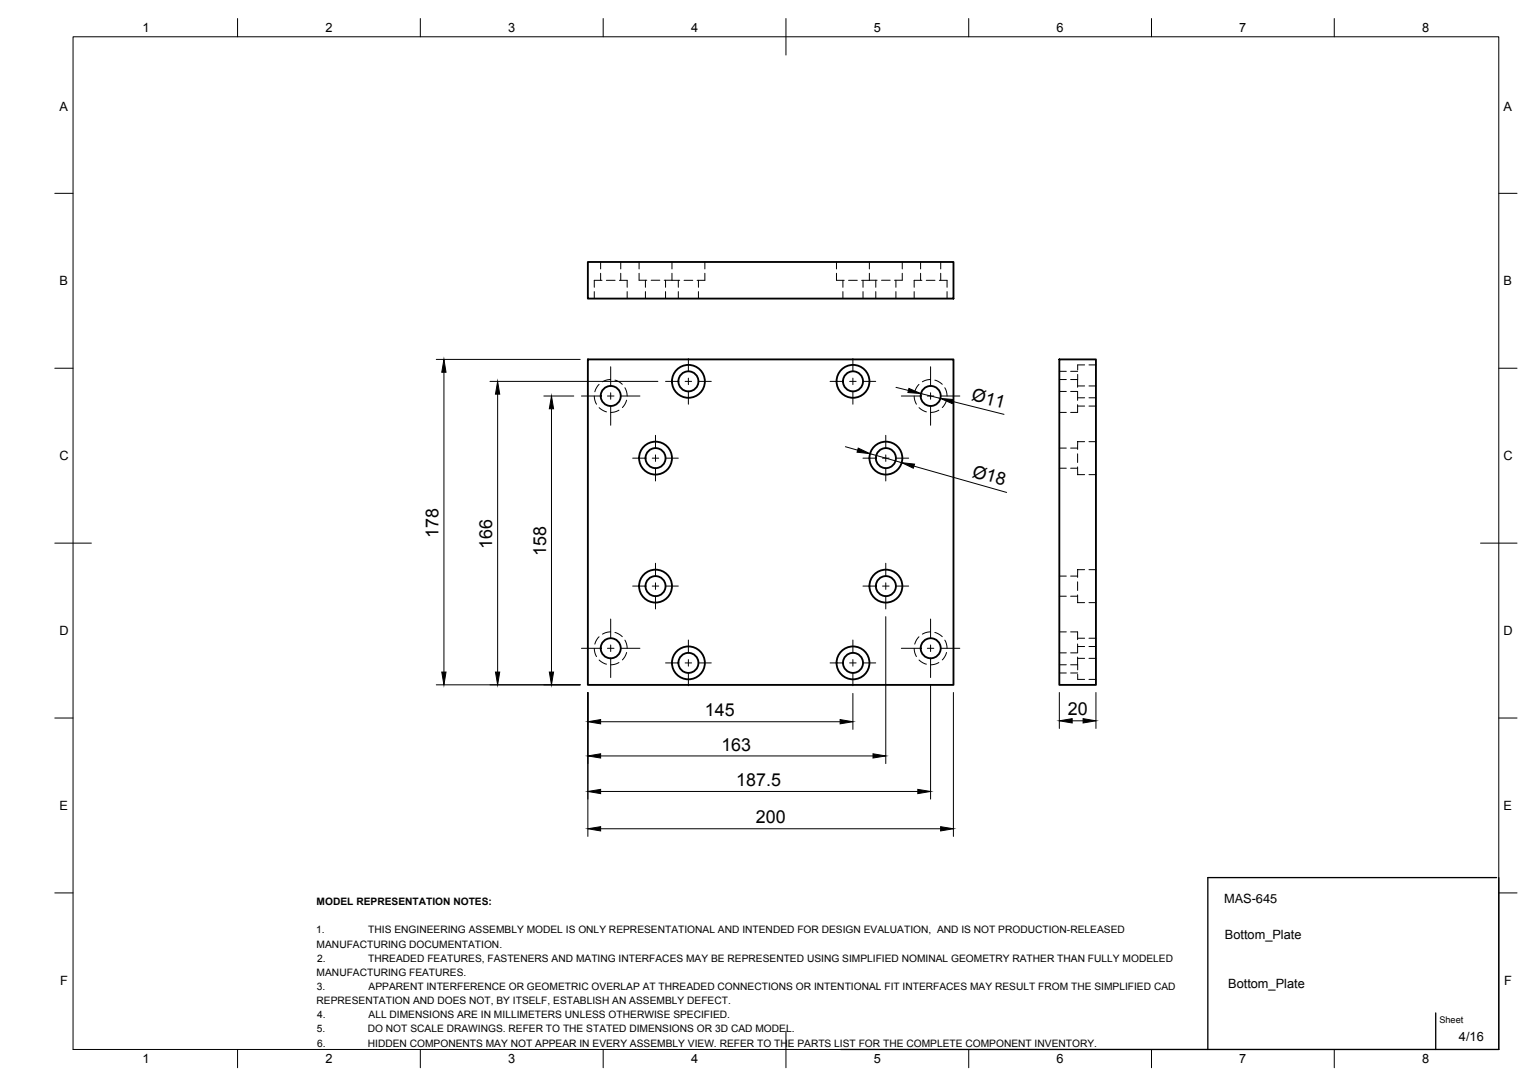
ISO-10303-21;
HEADER;
FILE_DESCRIPTION((''),'2;1');
FILE_NAME('Bottom_Plate.step','2026-10-09T10:54:55-07:00',(''),(''),'','','');
FILE_SCHEMA (('AUTOMOTIVE_DESIGN { 1 0 10303 214 3 1 1 }'));
ENDSEC;
DATA;
#10=MECHANICAL_DESIGN_GEOMETRIC_PRESENTATION_REPRESENTATION('',(#596),#63824);
#566=SHAPE_REPRESENTATION_RELATIONSHIP('SRR','None',#63880,#581) ;
#581=ADVANCED_BREP_SHAPE_REPRESENTATION('',(#611),#63810) ;
#596=STYLED_ITEM('',(#63963),#611) ;
#611=MANIFOLD_SOLID_BREP('Body1',#15495) ;
#651=FACE_BOUND('',#2476,.T.) ;
#652=FACE_BOUND('',#2480,.T.) ;
#653=FACE_BOUND('',#2484,.T.) ;
#654=FACE_BOUND('',#2488,.T.) ;
#655=FACE_BOUND('',#2492,.T.) ;
#656=FACE_BOUND('',#2496,.T.) ;
#657=FACE_BOUND('',#2500,.T.) ;
#658=FACE_BOUND('',#2504,.T.) ;
#659=FACE_BOUND('',#2508,.T.) ;
#660=FACE_BOUND('',#2512,.T.) ;
#661=FACE_BOUND('',#2516,.T.) ;
#662=FACE_BOUND('',#2520,.T.) ;
#663=FACE_BOUND('',#2524,.T.) ;
#664=FACE_BOUND('',#2525,.T.) ;
#665=FACE_BOUND('',#2526,.T.) ;
#666=FACE_BOUND('',#2527,.T.) ;
#667=FACE_BOUND('',#2528,.T.) ;
#668=FACE_BOUND('',#2529,.T.) ;
#669=FACE_BOUND('',#2530,.T.) ;
#670=FACE_BOUND('',#2531,.T.) ;
#671=FACE_BOUND('',#2532,.T.) ;
#672=FACE_BOUND('',#2533,.T.) ;
#673=FACE_BOUND('',#2534,.T.) ;
#674=FACE_BOUND('',#2535,.T.) ;
#675=FACE_BOUND('',#2538,.T.) ;
#676=FACE_BOUND('',#2539,.T.) ;
#677=FACE_BOUND('',#2540,.T.) ;
#678=FACE_BOUND('',#2541,.T.) ;
#679=FACE_BOUND('',#2542,.T.) ;
#680=FACE_BOUND('',#2543,.T.) ;
#681=FACE_BOUND('',#2544,.T.) ;
#682=FACE_BOUND('',#2545,.T.) ;
#683=FACE_BOUND('',#2546,.T.) ;
#684=FACE_BOUND('',#2547,.T.) ;
#685=FACE_BOUND('',#2548,.T.) ;
#686=FACE_BOUND('',#2549,.T.) ;
#842=PLANE('',#15763) ;
#843=PLANE('',#15770) ;
#844=PLANE('',#15777) ;
#845=PLANE('',#15784) ;
#846=PLANE('',#15791) ;
#847=PLANE('',#15798) ;
#848=PLANE('',#15805) ;
#849=PLANE('',#15812) ;
#850=PLANE('',#15819) ;
#851=PLANE('',#15826) ;
#852=PLANE('',#15833) ;
#853=PLANE('',#15840) ;
#854=PLANE('',#15847) ;
#855=PLANE('',#15848) ;
#856=PLANE('',#15849) ;
#857=PLANE('',#15850) ;
#858=PLANE('',#15851) ;
#859=PLANE('',#15852) ;
#1137=CYLINDRICAL_SURFACE('',#15766,9.) ;
#1138=CYLINDRICAL_SURFACE('',#15768,5.5) ;
#1139=CYLINDRICAL_SURFACE('',#15773,9.) ;
#1140=CYLINDRICAL_SURFACE('',#15775,5.5) ;
#1141=CYLINDRICAL_SURFACE('',#15780,9.) ;
#1142=CYLINDRICAL_SURFACE('',#15782,5.5) ;
#1143=CYLINDRICAL_SURFACE('',#15787,9.) ;
#1144=CYLINDRICAL_SURFACE('',#15789,5.5) ;
#1145=CYLINDRICAL_SURFACE('',#15794,9.) ;
#1146=CYLINDRICAL_SURFACE('',#15796,5.5) ;
#1147=CYLINDRICAL_SURFACE('',#15801,9.) ;
#1148=CYLINDRICAL_SURFACE('',#15803,5.5) ;
#1149=CYLINDRICAL_SURFACE('',#15808,9.) ;
#1150=CYLINDRICAL_SURFACE('',#15810,5.5) ;
#1151=CYLINDRICAL_SURFACE('',#15815,9.) ;
#1152=CYLINDRICAL_SURFACE('',#15817,5.5) ;
#1153=CYLINDRICAL_SURFACE('',#15822,9.) ;
#1154=CYLINDRICAL_SURFACE('',#15824,5.5) ;
#1155=CYLINDRICAL_SURFACE('',#15829,9.) ;
#1156=CYLINDRICAL_SURFACE('',#15831,5.5) ;
#1157=CYLINDRICAL_SURFACE('',#15836,9.) ;
#1158=CYLINDRICAL_SURFACE('',#15838,5.5) ;
#1159=CYLINDRICAL_SURFACE('',#15843,9.) ;
#1160=CYLINDRICAL_SURFACE('',#15845,5.5) ;
#1588=FACE_OUTER_BOUND('',#2475,.T.) ;
#1589=FACE_OUTER_BOUND('',#2477,.T.) ;
#1590=FACE_OUTER_BOUND('',#2478,.T.) ;
#1591=FACE_OUTER_BOUND('',#2479,.T.) ;
#1592=FACE_OUTER_BOUND('',#2481,.T.) ;
#1593=FACE_OUTER_BOUND('',#2482,.T.) ;
#1594=FACE_OUTER_BOUND('',#2483,.T.) ;
#1595=FACE_OUTER_BOUND('',#2485,.T.) ;
#1596=FACE_OUTER_BOUND('',#2486,.T.) ;
#1597=FACE_OUTER_BOUND('',#2487,.T.) ;
#1598=FACE_OUTER_BOUND('',#2489,.T.) ;
#1599=FACE_OUTER_BOUND('',#2490,.T.) ;
#1600=FACE_OUTER_BOUND('',#2491,.T.) ;
#1601=FACE_OUTER_BOUND('',#2493,.T.) ;
#1602=FACE_OUTER_BOUND('',#2494,.T.) ;
#1603=FACE_OUTER_BOUND('',#2495,.T.) ;
#1604=FACE_OUTER_BOUND('',#2497,.T.) ;
#1605=FACE_OUTER_BOUND('',#2498,.T.) ;
#1606=FACE_OUTER_BOUND('',#2499,.T.) ;
#1607=FACE_OUTER_BOUND('',#2501,.T.) ;
#1608=FACE_OUTER_BOUND('',#2502,.T.) ;
#1609=FACE_OUTER_BOUND('',#2503,.T.) ;
#1610=FACE_OUTER_BOUND('',#2505,.T.) ;
#1611=FACE_OUTER_BOUND('',#2506,.T.) ;
#1612=FACE_OUTER_BOUND('',#2507,.T.) ;
#1613=FACE_OUTER_BOUND('',#2509,.T.) ;
#1614=FACE_OUTER_BOUND('',#2510,.T.) ;
#1615=FACE_OUTER_BOUND('',#2511,.T.) ;
#1616=FACE_OUTER_BOUND('',#2513,.T.) ;
#1617=FACE_OUTER_BOUND('',#2514,.T.) ;
#1618=FACE_OUTER_BOUND('',#2515,.T.) ;
#1619=FACE_OUTER_BOUND('',#2517,.T.) ;
#1620=FACE_OUTER_BOUND('',#2518,.T.) ;
#1621=FACE_OUTER_BOUND('',#2519,.T.) ;
#1622=FACE_OUTER_BOUND('',#2521,.T.) ;
#1623=FACE_OUTER_BOUND('',#2522,.T.) ;
#1624=FACE_OUTER_BOUND('',#2523,.T.) ;
#1625=FACE_OUTER_BOUND('',#2536,.T.) ;
#1626=FACE_OUTER_BOUND('',#2537,.T.) ;
#1627=FACE_OUTER_BOUND('',#2550,.T.) ;
#1628=FACE_OUTER_BOUND('',#2551,.T.) ;
#1629=FACE_OUTER_BOUND('',#2552,.T.) ;
#2475=EDGE_LOOP('',(#9976)) ;
#2476=EDGE_LOOP('',(#9977)) ;
#2477=EDGE_LOOP('',(#9978,#9979,#9980,#9981)) ;
#2478=EDGE_LOOP('',(#9982,#9983,#9984,#9985)) ;
#2479=EDGE_LOOP('',(#9986)) ;
#2480=EDGE_LOOP('',(#9987)) ;
#2481=EDGE_LOOP('',(#9988,#9989,#9990,#9991)) ;
#2482=EDGE_LOOP('',(#9992,#9993,#9994,#9995)) ;
#2483=EDGE_LOOP('',(#9996)) ;
#2484=EDGE_LOOP('',(#9997)) ;
#2485=EDGE_LOOP('',(#9998,#9999,#10000,#10001)) ;
#2486=EDGE_LOOP('',(#10002,#10003,#10004,#10005)) ;
#2487=EDGE_LOOP('',(#10006)) ;
#2488=EDGE_LOOP('',(#10007)) ;
#2489=EDGE_LOOP('',(#10008,#10009,#10010,#10011)) ;
#2490=EDGE_LOOP('',(#10012,#10013,#10014,#10015)) ;
#2491=EDGE_LOOP('',(#10016)) ;
#2492=EDGE_LOOP('',(#10017)) ;
#2493=EDGE_LOOP('',(#10018,#10019,#10020,#10021)) ;
#2494=EDGE_LOOP('',(#10022,#10023,#10024,#10025)) ;
#2495=EDGE_LOOP('',(#10026)) ;
#2496=EDGE_LOOP('',(#10027)) ;
#2497=EDGE_LOOP('',(#10028,#10029,#10030,#10031)) ;
#2498=EDGE_LOOP('',(#10032,#10033,#10034,#10035)) ;
#2499=EDGE_LOOP('',(#10036)) ;
#2500=EDGE_LOOP('',(#10037)) ;
#2501=EDGE_LOOP('',(#10038,#10039,#10040,#10041)) ;
#2502=EDGE_LOOP('',(#10042,#10043,#10044,#10045)) ;
#2503=EDGE_LOOP('',(#10046)) ;
#2504=EDGE_LOOP('',(#10047)) ;
#2505=EDGE_LOOP('',(#10048,#10049,#10050,#10051)) ;
#2506=EDGE_LOOP('',(#10052,#10053,#10054,#10055)) ;
#2507=EDGE_LOOP('',(#10056)) ;
#2508=EDGE_LOOP('',(#10057)) ;
#2509=EDGE_LOOP('',(#10058,#10059,#10060,#10061)) ;
#2510=EDGE_LOOP('',(#10062,#10063,#10064,#10065)) ;
#2511=EDGE_LOOP('',(#10066)) ;
#2512=EDGE_LOOP('',(#10067)) ;
#2513=EDGE_LOOP('',(#10068,#10069,#10070,#10071)) ;
#2514=EDGE_LOOP('',(#10072,#10073,#10074,#10075)) ;
#2515=EDGE_LOOP('',(#10076)) ;
#2516=EDGE_LOOP('',(#10077)) ;
#2517=EDGE_LOOP('',(#10078,#10079,#10080,#10081)) ;
#2518=EDGE_LOOP('',(#10082,#10083,#10084,#10085)) ;
#2519=EDGE_LOOP('',(#10086)) ;
#2520=EDGE_LOOP('',(#10087)) ;
#2521=EDGE_LOOP('',(#10088,#10089,#10090,#10091)) ;
#2522=EDGE_LOOP('',(#10092,#10093,#10094,#10095)) ;
#2523=EDGE_LOOP('',(#10096,#10097,#10098,#10099)) ;
#2524=EDGE_LOOP('',(#10100)) ;
#2525=EDGE_LOOP('',(#10101)) ;
#2526=EDGE_LOOP('',(#10102)) ;
#2527=EDGE_LOOP('',(#10103)) ;
#2528=EDGE_LOOP('',(#10104)) ;
#2529=EDGE_LOOP('',(#10105)) ;
#2530=EDGE_LOOP('',(#10106)) ;
#2531=EDGE_LOOP('',(#10107)) ;
#2532=EDGE_LOOP('',(#10108)) ;
#2533=EDGE_LOOP('',(#10109)) ;
#2534=EDGE_LOOP('',(#10110)) ;
#2535=EDGE_LOOP('',(#10111)) ;
#2536=EDGE_LOOP('',(#10112,#10113,#10114,#10115)) ;
#2537=EDGE_LOOP('',(#10116,#10117,#10118,#10119)) ;
#2538=EDGE_LOOP('',(#10120)) ;
#2539=EDGE_LOOP('',(#10121)) ;
#2540=EDGE_LOOP('',(#10122)) ;
#2541=EDGE_LOOP('',(#10123)) ;
#2542=EDGE_LOOP('',(#10124)) ;
#2543=EDGE_LOOP('',(#10125)) ;
#2544=EDGE_LOOP('',(#10126)) ;
#2545=EDGE_LOOP('',(#10127)) ;
#2546=EDGE_LOOP('',(#10128)) ;
#2547=EDGE_LOOP('',(#10129)) ;
#2548=EDGE_LOOP('',(#10130)) ;
#2549=EDGE_LOOP('',(#10131)) ;
#2550=EDGE_LOOP('',(#10132,#10133,#10134,#10135)) ;
#2551=EDGE_LOOP('',(#10136,#10137,#10138,#10139)) ;
#2552=EDGE_LOOP('',(#10140,#10141,#10142,#10143)) ;
#3516=CIRCLE('',#15764,9.) ;
#3517=CIRCLE('',#15765,5.5) ;
#3518=CIRCLE('',#15767,9.) ;
#3519=CIRCLE('',#15769,5.5) ;
#3520=CIRCLE('',#15771,9.) ;
#3521=CIRCLE('',#15772,5.5) ;
#3522=CIRCLE('',#15774,9.) ;
#3523=CIRCLE('',#15776,5.5) ;
#3524=CIRCLE('',#15778,9.) ;
#3525=CIRCLE('',#15779,5.5) ;
#3526=CIRCLE('',#15781,9.) ;
#3527=CIRCLE('',#15783,5.5) ;
#3528=CIRCLE('',#15785,9.) ;
#3529=CIRCLE('',#15786,5.5) ;
#3530=CIRCLE('',#15788,9.) ;
#3531=CIRCLE('',#15790,5.5) ;
#3532=CIRCLE('',#15792,9.) ;
#3533=CIRCLE('',#15793,5.5) ;
#3534=CIRCLE('',#15795,9.) ;
#3535=CIRCLE('',#15797,5.5) ;
#3536=CIRCLE('',#15799,9.) ;
#3537=CIRCLE('',#15800,5.5) ;
#3538=CIRCLE('',#15802,9.) ;
#3539=CIRCLE('',#15804,5.5) ;
#3540=CIRCLE('',#15806,9.) ;
#3541=CIRCLE('',#15807,5.5) ;
#3542=CIRCLE('',#15809,9.) ;
#3543=CIRCLE('',#15811,5.5) ;
#3544=CIRCLE('',#15813,9.) ;
#3545=CIRCLE('',#15814,5.5) ;
#3546=CIRCLE('',#15816,9.) ;
#3547=CIRCLE('',#15818,5.5) ;
#3548=CIRCLE('',#15820,9.) ;
#3549=CIRCLE('',#15821,5.5) ;
#3550=CIRCLE('',#15823,9.) ;
#3551=CIRCLE('',#15825,5.5) ;
#3552=CIRCLE('',#15827,9.) ;
#3553=CIRCLE('',#15828,5.5) ;
#3554=CIRCLE('',#15830,9.) ;
#3555=CIRCLE('',#15832,5.5) ;
#3556=CIRCLE('',#15834,9.) ;
#3557=CIRCLE('',#15835,5.5) ;
#3558=CIRCLE('',#15837,9.) ;
#3559=CIRCLE('',#15839,5.5) ;
#3560=CIRCLE('',#15841,9.) ;
#3561=CIRCLE('',#15842,5.5) ;
#3562=CIRCLE('',#15844,9.) ;
#3563=CIRCLE('',#15846,5.5) ;
#4735=LINE('',#23215,#5391) ;
#4736=LINE('',#23218,#5392) ;
#4737=LINE('',#23228,#5393) ;
#4738=LINE('',#23231,#5394) ;
#4739=LINE('',#23241,#5395) ;
#4740=LINE('',#23244,#5396) ;
#4741=LINE('',#23254,#5397) ;
#4742=LINE('',#23257,#5398) ;
#4743=LINE('',#23267,#5399) ;
#4744=LINE('',#23270,#5400) ;
#4745=LINE('',#23280,#5401) ;
#4746=LINE('',#23283,#5402) ;
#4747=LINE('',#23293,#5403) ;
#4748=LINE('',#23296,#5404) ;
#4749=LINE('',#23306,#5405) ;
#4750=LINE('',#23309,#5406) ;
#4751=LINE('',#23319,#5407) ;
#4752=LINE('',#23322,#5408) ;
#4753=LINE('',#23332,#5409) ;
#4754=LINE('',#23335,#5410) ;
#4755=LINE('',#23345,#5411) ;
#4756=LINE('',#23348,#5412) ;
#4757=LINE('',#23358,#5413) ;
#4758=LINE('',#23361,#5414) ;
#4759=LINE('',#23366,#5415) ;
#4760=LINE('',#23368,#5416) ;
#4761=LINE('',#23370,#5417) ;
#4762=LINE('',#23371,#5418) ;
#4763=LINE('',#23374,#5419) ;
#4764=LINE('',#23376,#5420) ;
#4765=LINE('',#23377,#5421) ;
#4766=LINE('',#23380,#5422) ;
#4767=LINE('',#23382,#5423) ;
#4768=LINE('',#23383,#5424) ;
#4769=LINE('',#23385,#5425) ;
#4770=LINE('',#23386,#5426) ;
#5391=VECTOR('',#18133,9.) ;
#5392=VECTOR('',#18136,5.5) ;
#5393=VECTOR('',#18149,9.) ;
#5394=VECTOR('',#18152,5.5) ;
#5395=VECTOR('',#18165,9.) ;
#5396=VECTOR('',#18168,5.5) ;
#5397=VECTOR('',#18181,9.) ;
#5398=VECTOR('',#18184,5.5) ;
#5399=VECTOR('',#18197,9.) ;
#5400=VECTOR('',#18200,5.5) ;
#5401=VECTOR('',#18213,9.) ;
#5402=VECTOR('',#18216,5.5) ;
#5403=VECTOR('',#18229,9.) ;
#5404=VECTOR('',#18232,5.5) ;
#5405=VECTOR('',#18245,9.) ;
#5406=VECTOR('',#18248,5.5) ;
#5407=VECTOR('',#18261,9.) ;
#5408=VECTOR('',#18264,5.5) ;
#5409=VECTOR('',#18277,9.) ;
#5410=VECTOR('',#18280,5.5) ;
#5411=VECTOR('',#18293,9.) ;
#5412=VECTOR('',#18296,5.5) ;
#5413=VECTOR('',#18309,9.) ;
#5414=VECTOR('',#18312,5.5) ;
#5415=VECTOR('',#18317,10.) ;
#5416=VECTOR('',#18318,10.) ;
#5417=VECTOR('',#18319,10.) ;
#5418=VECTOR('',#18320,10.) ;
#5419=VECTOR('',#18323,10.) ;
#5420=VECTOR('',#18324,10.) ;
#5421=VECTOR('',#18325,10.) ;
#5422=VECTOR('',#18328,10.) ;
#5423=VECTOR('',#18329,10.) ;
#5424=VECTOR('',#18330,10.) ;
#5425=VECTOR('',#18333,10.) ;
#5426=VECTOR('',#18334,10.) ;
#6064=VERTEX_POINT('',#23208) ;
#6065=VERTEX_POINT('',#23210) ;
#6066=VERTEX_POINT('',#23213) ;
#6067=VERTEX_POINT('',#23217) ;
#6068=VERTEX_POINT('',#23221) ;
#6069=VERTEX_POINT('',#23223) ;
#6070=VERTEX_POINT('',#23226) ;
#6071=VERTEX_POINT('',#23230) ;
#6072=VERTEX_POINT('',#23234) ;
#6073=VERTEX_POINT('',#23236) ;
#6074=VERTEX_POINT('',#23239) ;
#6075=VERTEX_POINT('',#23243) ;
#6076=VERTEX_POINT('',#23247) ;
#6077=VERTEX_POINT('',#23249) ;
#6078=VERTEX_POINT('',#23252) ;
#6079=VERTEX_POINT('',#23256) ;
#6080=VERTEX_POINT('',#23260) ;
#6081=VERTEX_POINT('',#23262) ;
#6082=VERTEX_POINT('',#23265) ;
#6083=VERTEX_POINT('',#23269) ;
#6084=VERTEX_POINT('',#23273) ;
#6085=VERTEX_POINT('',#23275) ;
#6086=VERTEX_POINT('',#23278) ;
#6087=VERTEX_POINT('',#23282) ;
#6088=VERTEX_POINT('',#23286) ;
#6089=VERTEX_POINT('',#23288) ;
#6090=VERTEX_POINT('',#23291) ;
#6091=VERTEX_POINT('',#23295) ;
#6092=VERTEX_POINT('',#23299) ;
#6093=VERTEX_POINT('',#23301) ;
#6094=VERTEX_POINT('',#23304) ;
#6095=VERTEX_POINT('',#23308) ;
#6096=VERTEX_POINT('',#23312) ;
#6097=VERTEX_POINT('',#23314) ;
#6098=VERTEX_POINT('',#23317) ;
#6099=VERTEX_POINT('',#23321) ;
#6100=VERTEX_POINT('',#23325) ;
#6101=VERTEX_POINT('',#23327) ;
#6102=VERTEX_POINT('',#23330) ;
#6103=VERTEX_POINT('',#23334) ;
#6104=VERTEX_POINT('',#23338) ;
#6105=VERTEX_POINT('',#23340) ;
#6106=VERTEX_POINT('',#23343) ;
#6107=VERTEX_POINT('',#23347) ;
#6108=VERTEX_POINT('',#23351) ;
#6109=VERTEX_POINT('',#23353) ;
#6110=VERTEX_POINT('',#23356) ;
#6111=VERTEX_POINT('',#23360) ;
#6112=VERTEX_POINT('',#23364) ;
#6113=VERTEX_POINT('',#23365) ;
#6114=VERTEX_POINT('',#23367) ;
#6115=VERTEX_POINT('',#23369) ;
#6116=VERTEX_POINT('',#23373) ;
#6117=VERTEX_POINT('',#23375) ;
#6118=VERTEX_POINT('',#23379) ;
#6119=VERTEX_POINT('',#23381) ;
#7542=EDGE_CURVE('',#6064,#6064,#3516,.T.) ;
#7543=EDGE_CURVE('',#6065,#6065,#3517,.T.) ;
#7544=EDGE_CURVE('',#6066,#6066,#3518,.T.) ;
#7545=EDGE_CURVE('',#6066,#6064,#4735,.T.) ;
#7546=EDGE_CURVE('',#6065,#6067,#4736,.T.) ;
#7547=EDGE_CURVE('',#6067,#6067,#3519,.T.) ;
#7548=EDGE_CURVE('',#6068,#6068,#3520,.T.) ;
#7549=EDGE_CURVE('',#6069,#6069,#3521,.T.) ;
#7550=EDGE_CURVE('',#6070,#6070,#3522,.T.) ;
#7551=EDGE_CURVE('',#6070,#6068,#4737,.T.) ;
#7552=EDGE_CURVE('',#6069,#6071,#4738,.T.) ;
#7553=EDGE_CURVE('',#6071,#6071,#3523,.T.) ;
#7554=EDGE_CURVE('',#6072,#6072,#3524,.T.) ;
#7555=EDGE_CURVE('',#6073,#6073,#3525,.T.) ;
#7556=EDGE_CURVE('',#6074,#6074,#3526,.T.) ;
#7557=EDGE_CURVE('',#6074,#6072,#4739,.T.) ;
#7558=EDGE_CURVE('',#6073,#6075,#4740,.T.) ;
#7559=EDGE_CURVE('',#6075,#6075,#3527,.T.) ;
#7560=EDGE_CURVE('',#6076,#6076,#3528,.T.) ;
#7561=EDGE_CURVE('',#6077,#6077,#3529,.T.) ;
#7562=EDGE_CURVE('',#6078,#6078,#3530,.T.) ;
#7563=EDGE_CURVE('',#6078,#6076,#4741,.T.) ;
#7564=EDGE_CURVE('',#6077,#6079,#4742,.T.) ;
#7565=EDGE_CURVE('',#6079,#6079,#3531,.T.) ;
#7566=EDGE_CURVE('',#6080,#6080,#3532,.T.) ;
#7567=EDGE_CURVE('',#6081,#6081,#3533,.T.) ;
#7568=EDGE_CURVE('',#6082,#6082,#3534,.T.) ;
#7569=EDGE_CURVE('',#6082,#6080,#4743,.T.) ;
#7570=EDGE_CURVE('',#6081,#6083,#4744,.T.) ;
#7571=EDGE_CURVE('',#6083,#6083,#3535,.T.) ;
#7572=EDGE_CURVE('',#6084,#6084,#3536,.T.) ;
#7573=EDGE_CURVE('',#6085,#6085,#3537,.T.) ;
#7574=EDGE_CURVE('',#6086,#6086,#3538,.T.) ;
#7575=EDGE_CURVE('',#6086,#6084,#4745,.T.) ;
#7576=EDGE_CURVE('',#6085,#6087,#4746,.T.) ;
#7577=EDGE_CURVE('',#6087,#6087,#3539,.T.) ;
#7578=EDGE_CURVE('',#6088,#6088,#3540,.T.) ;
#7579=EDGE_CURVE('',#6089,#6089,#3541,.T.) ;
#7580=EDGE_CURVE('',#6090,#6090,#3542,.T.) ;
#7581=EDGE_CURVE('',#6090,#6088,#4747,.T.) ;
#7582=EDGE_CURVE('',#6089,#6091,#4748,.T.) ;
#7583=EDGE_CURVE('',#6091,#6091,#3543,.T.) ;
#7584=EDGE_CURVE('',#6092,#6092,#3544,.T.) ;
#7585=EDGE_CURVE('',#6093,#6093,#3545,.T.) ;
#7586=EDGE_CURVE('',#6094,#6094,#3546,.T.) ;
#7587=EDGE_CURVE('',#6094,#6092,#4749,.T.) ;
#7588=EDGE_CURVE('',#6093,#6095,#4750,.T.) ;
#7589=EDGE_CURVE('',#6095,#6095,#3547,.T.) ;
#7590=EDGE_CURVE('',#6096,#6096,#3548,.T.) ;
#7591=EDGE_CURVE('',#6097,#6097,#3549,.T.) ;
#7592=EDGE_CURVE('',#6098,#6098,#3550,.T.) ;
#7593=EDGE_CURVE('',#6098,#6096,#4751,.T.) ;
#7594=EDGE_CURVE('',#6097,#6099,#4752,.T.) ;
#7595=EDGE_CURVE('',#6099,#6099,#3551,.T.) ;
#7596=EDGE_CURVE('',#6100,#6100,#3552,.T.) ;
#7597=EDGE_CURVE('',#6101,#6101,#3553,.T.) ;
#7598=EDGE_CURVE('',#6102,#6102,#3554,.T.) ;
#7599=EDGE_CURVE('',#6102,#6100,#4753,.T.) ;
#7600=EDGE_CURVE('',#6101,#6103,#4754,.T.) ;
#7601=EDGE_CURVE('',#6103,#6103,#3555,.T.) ;
#7602=EDGE_CURVE('',#6104,#6104,#3556,.T.) ;
#7603=EDGE_CURVE('',#6105,#6105,#3557,.T.) ;
#7604=EDGE_CURVE('',#6106,#6106,#3558,.T.) ;
#7605=EDGE_CURVE('',#6106,#6104,#4755,.T.) ;
#7606=EDGE_CURVE('',#6105,#6107,#4756,.T.) ;
#7607=EDGE_CURVE('',#6107,#6107,#3559,.T.) ;
#7608=EDGE_CURVE('',#6108,#6108,#3560,.T.) ;
#7609=EDGE_CURVE('',#6109,#6109,#3561,.T.) ;
#7610=EDGE_CURVE('',#6110,#6110,#3562,.T.) ;
#7611=EDGE_CURVE('',#6110,#6108,#4757,.T.) ;
#7612=EDGE_CURVE('',#6109,#6111,#4758,.T.) ;
#7613=EDGE_CURVE('',#6111,#6111,#3563,.T.) ;
#7614=EDGE_CURVE('',#6112,#6113,#4759,.T.) ;
#7615=EDGE_CURVE('',#6114,#6113,#4760,.T.) ;
#7616=EDGE_CURVE('',#6114,#6115,#4761,.T.) ;
#7617=EDGE_CURVE('',#6115,#6112,#4762,.T.) ;
#7618=EDGE_CURVE('',#6113,#6116,#4763,.T.) ;
#7619=EDGE_CURVE('',#6117,#6116,#4764,.T.) ;
#7620=EDGE_CURVE('',#6117,#6114,#4765,.T.) ;
#7621=EDGE_CURVE('',#6116,#6118,#4766,.T.) ;
#7622=EDGE_CURVE('',#6119,#6118,#4767,.T.) ;
#7623=EDGE_CURVE('',#6119,#6117,#4768,.T.) ;
#7624=EDGE_CURVE('',#6118,#6112,#4769,.T.) ;
#7625=EDGE_CURVE('',#6115,#6119,#4770,.T.) ;
#9976=ORIENTED_EDGE('',*,*,#7542,.F.) ;
#9977=ORIENTED_EDGE('',*,*,#7543,.T.) ;
#9978=ORIENTED_EDGE('',*,*,#7544,.F.) ;
#9979=ORIENTED_EDGE('',*,*,#7545,.T.) ;
#9980=ORIENTED_EDGE('',*,*,#7542,.T.) ;
#9981=ORIENTED_EDGE('',*,*,#7545,.F.) ;
#9982=ORIENTED_EDGE('',*,*,#7543,.F.) ;
#9983=ORIENTED_EDGE('',*,*,#7546,.T.) ;
#9984=ORIENTED_EDGE('',*,*,#7547,.F.) ;
#9985=ORIENTED_EDGE('',*,*,#7546,.F.) ;
#9986=ORIENTED_EDGE('',*,*,#7548,.F.) ;
#9987=ORIENTED_EDGE('',*,*,#7549,.T.) ;
#9988=ORIENTED_EDGE('',*,*,#7550,.F.) ;
#9989=ORIENTED_EDGE('',*,*,#7551,.T.) ;
#9990=ORIENTED_EDGE('',*,*,#7548,.T.) ;
#9991=ORIENTED_EDGE('',*,*,#7551,.F.) ;
#9992=ORIENTED_EDGE('',*,*,#7549,.F.) ;
#9993=ORIENTED_EDGE('',*,*,#7552,.T.) ;
#9994=ORIENTED_EDGE('',*,*,#7553,.F.) ;
#9995=ORIENTED_EDGE('',*,*,#7552,.F.) ;
#9996=ORIENTED_EDGE('',*,*,#7554,.F.) ;
#9997=ORIENTED_EDGE('',*,*,#7555,.T.) ;
#9998=ORIENTED_EDGE('',*,*,#7556,.F.) ;
#9999=ORIENTED_EDGE('',*,*,#7557,.T.) ;
#10000=ORIENTED_EDGE('',*,*,#7554,.T.) ;
#10001=ORIENTED_EDGE('',*,*,#7557,.F.) ;
#10002=ORIENTED_EDGE('',*,*,#7555,.F.) ;
#10003=ORIENTED_EDGE('',*,*,#7558,.T.) ;
#10004=ORIENTED_EDGE('',*,*,#7559,.F.) ;
#10005=ORIENTED_EDGE('',*,*,#7558,.F.) ;
#10006=ORIENTED_EDGE('',*,*,#7560,.F.) ;
#10007=ORIENTED_EDGE('',*,*,#7561,.T.) ;
#10008=ORIENTED_EDGE('',*,*,#7562,.F.) ;
#10009=ORIENTED_EDGE('',*,*,#7563,.T.) ;
#10010=ORIENTED_EDGE('',*,*,#7560,.T.) ;
#10011=ORIENTED_EDGE('',*,*,#7563,.F.) ;
#10012=ORIENTED_EDGE('',*,*,#7561,.F.) ;
#10013=ORIENTED_EDGE('',*,*,#7564,.T.) ;
#10014=ORIENTED_EDGE('',*,*,#7565,.F.) ;
#10015=ORIENTED_EDGE('',*,*,#7564,.F.) ;
#10016=ORIENTED_EDGE('',*,*,#7566,.F.) ;
#10017=ORIENTED_EDGE('',*,*,#7567,.T.) ;
#10018=ORIENTED_EDGE('',*,*,#7568,.F.) ;
#10019=ORIENTED_EDGE('',*,*,#7569,.T.) ;
#10020=ORIENTED_EDGE('',*,*,#7566,.T.) ;
#10021=ORIENTED_EDGE('',*,*,#7569,.F.) ;
#10022=ORIENTED_EDGE('',*,*,#7567,.F.) ;
#10023=ORIENTED_EDGE('',*,*,#7570,.T.) ;
#10024=ORIENTED_EDGE('',*,*,#7571,.F.) ;
#10025=ORIENTED_EDGE('',*,*,#7570,.F.) ;
#10026=ORIENTED_EDGE('',*,*,#7572,.F.) ;
#10027=ORIENTED_EDGE('',*,*,#7573,.T.) ;
#10028=ORIENTED_EDGE('',*,*,#7574,.F.) ;
#10029=ORIENTED_EDGE('',*,*,#7575,.T.) ;
#10030=ORIENTED_EDGE('',*,*,#7572,.T.) ;
#10031=ORIENTED_EDGE('',*,*,#7575,.F.) ;
#10032=ORIENTED_EDGE('',*,*,#7573,.F.) ;
#10033=ORIENTED_EDGE('',*,*,#7576,.T.) ;
#10034=ORIENTED_EDGE('',*,*,#7577,.F.) ;
#10035=ORIENTED_EDGE('',*,*,#7576,.F.) ;
#10036=ORIENTED_EDGE('',*,*,#7578,.F.) ;
#10037=ORIENTED_EDGE('',*,*,#7579,.T.) ;
#10038=ORIENTED_EDGE('',*,*,#7580,.F.) ;
#10039=ORIENTED_EDGE('',*,*,#7581,.T.) ;
#10040=ORIENTED_EDGE('',*,*,#7578,.T.) ;
#10041=ORIENTED_EDGE('',*,*,#7581,.F.) ;
#10042=ORIENTED_EDGE('',*,*,#7579,.F.) ;
#10043=ORIENTED_EDGE('',*,*,#7582,.T.) ;
#10044=ORIENTED_EDGE('',*,*,#7583,.F.) ;
#10045=ORIENTED_EDGE('',*,*,#7582,.F.) ;
#10046=ORIENTED_EDGE('',*,*,#7584,.F.) ;
#10047=ORIENTED_EDGE('',*,*,#7585,.T.) ;
#10048=ORIENTED_EDGE('',*,*,#7586,.F.) ;
#10049=ORIENTED_EDGE('',*,*,#7587,.T.) ;
#10050=ORIENTED_EDGE('',*,*,#7584,.T.) ;
#10051=ORIENTED_EDGE('',*,*,#7587,.F.) ;
#10052=ORIENTED_EDGE('',*,*,#7585,.F.) ;
#10053=ORIENTED_EDGE('',*,*,#7588,.T.) ;
#10054=ORIENTED_EDGE('',*,*,#7589,.F.) ;
#10055=ORIENTED_EDGE('',*,*,#7588,.F.) ;
#10056=ORIENTED_EDGE('',*,*,#7590,.F.) ;
#10057=ORIENTED_EDGE('',*,*,#7591,.T.) ;
#10058=ORIENTED_EDGE('',*,*,#7592,.F.) ;
#10059=ORIENTED_EDGE('',*,*,#7593,.T.) ;
#10060=ORIENTED_EDGE('',*,*,#7590,.T.) ;
#10061=ORIENTED_EDGE('',*,*,#7593,.F.) ;
#10062=ORIENTED_EDGE('',*,*,#7591,.F.) ;
#10063=ORIENTED_EDGE('',*,*,#7594,.T.) ;
#10064=ORIENTED_EDGE('',*,*,#7595,.F.) ;
#10065=ORIENTED_EDGE('',*,*,#7594,.F.) ;
#10066=ORIENTED_EDGE('',*,*,#7596,.F.) ;
#10067=ORIENTED_EDGE('',*,*,#7597,.T.) ;
#10068=ORIENTED_EDGE('',*,*,#7598,.F.) ;
#10069=ORIENTED_EDGE('',*,*,#7599,.T.) ;
#10070=ORIENTED_EDGE('',*,*,#7596,.T.) ;
#10071=ORIENTED_EDGE('',*,*,#7599,.F.) ;
#10072=ORIENTED_EDGE('',*,*,#7597,.F.) ;
#10073=ORIENTED_EDGE('',*,*,#7600,.T.) ;
#10074=ORIENTED_EDGE('',*,*,#7601,.F.) ;
#10075=ORIENTED_EDGE('',*,*,#7600,.F.) ;
#10076=ORIENTED_EDGE('',*,*,#7602,.F.) ;
#10077=ORIENTED_EDGE('',*,*,#7603,.T.) ;
#10078=ORIENTED_EDGE('',*,*,#7604,.F.) ;
#10079=ORIENTED_EDGE('',*,*,#7605,.T.) ;
#10080=ORIENTED_EDGE('',*,*,#7602,.T.) ;
#10081=ORIENTED_EDGE('',*,*,#7605,.F.) ;
#10082=ORIENTED_EDGE('',*,*,#7603,.F.) ;
#10083=ORIENTED_EDGE('',*,*,#7606,.T.) ;
#10084=ORIENTED_EDGE('',*,*,#7607,.F.) ;
#10085=ORIENTED_EDGE('',*,*,#7606,.F.) ;
#10086=ORIENTED_EDGE('',*,*,#7608,.F.) ;
#10087=ORIENTED_EDGE('',*,*,#7609,.T.) ;
#10088=ORIENTED_EDGE('',*,*,#7610,.F.) ;
#10089=ORIENTED_EDGE('',*,*,#7611,.T.) ;
#10090=ORIENTED_EDGE('',*,*,#7608,.T.) ;
#10091=ORIENTED_EDGE('',*,*,#7611,.F.) ;
#10092=ORIENTED_EDGE('',*,*,#7609,.F.) ;
#10093=ORIENTED_EDGE('',*,*,#7612,.T.) ;
#10094=ORIENTED_EDGE('',*,*,#7613,.F.) ;
#10095=ORIENTED_EDGE('',*,*,#7612,.F.) ;
#10096=ORIENTED_EDGE('',*,*,#7614,.T.) ;
#10097=ORIENTED_EDGE('',*,*,#7615,.F.) ;
#10098=ORIENTED_EDGE('',*,*,#7616,.T.) ;
#10099=ORIENTED_EDGE('',*,*,#7617,.T.) ;
#10100=ORIENTED_EDGE('',*,*,#7547,.T.) ;
#10101=ORIENTED_EDGE('',*,*,#7553,.T.) ;
#10102=ORIENTED_EDGE('',*,*,#7559,.T.) ;
#10103=ORIENTED_EDGE('',*,*,#7565,.T.) ;
#10104=ORIENTED_EDGE('',*,*,#7571,.T.) ;
#10105=ORIENTED_EDGE('',*,*,#7577,.T.) ;
#10106=ORIENTED_EDGE('',*,*,#7583,.T.) ;
#10107=ORIENTED_EDGE('',*,*,#7589,.T.) ;
#10108=ORIENTED_EDGE('',*,*,#7592,.T.) ;
#10109=ORIENTED_EDGE('',*,*,#7598,.T.) ;
#10110=ORIENTED_EDGE('',*,*,#7604,.T.) ;
#10111=ORIENTED_EDGE('',*,*,#7610,.T.) ;
#10112=ORIENTED_EDGE('',*,*,#7618,.T.) ;
#10113=ORIENTED_EDGE('',*,*,#7619,.F.) ;
#10114=ORIENTED_EDGE('',*,*,#7620,.T.) ;
#10115=ORIENTED_EDGE('',*,*,#7615,.T.) ;
#10116=ORIENTED_EDGE('',*,*,#7621,.T.) ;
#10117=ORIENTED_EDGE('',*,*,#7622,.F.) ;
#10118=ORIENTED_EDGE('',*,*,#7623,.T.) ;
#10119=ORIENTED_EDGE('',*,*,#7619,.T.) ;
#10120=ORIENTED_EDGE('',*,*,#7544,.T.) ;
#10121=ORIENTED_EDGE('',*,*,#7550,.T.) ;
#10122=ORIENTED_EDGE('',*,*,#7556,.T.) ;
#10123=ORIENTED_EDGE('',*,*,#7562,.T.) ;
#10124=ORIENTED_EDGE('',*,*,#7568,.T.) ;
#10125=ORIENTED_EDGE('',*,*,#7574,.T.) ;
#10126=ORIENTED_EDGE('',*,*,#7580,.T.) ;
#10127=ORIENTED_EDGE('',*,*,#7586,.T.) ;
#10128=ORIENTED_EDGE('',*,*,#7595,.T.) ;
#10129=ORIENTED_EDGE('',*,*,#7601,.T.) ;
#10130=ORIENTED_EDGE('',*,*,#7607,.T.) ;
#10131=ORIENTED_EDGE('',*,*,#7613,.T.) ;
#10132=ORIENTED_EDGE('',*,*,#7624,.T.) ;
#10133=ORIENTED_EDGE('',*,*,#7617,.F.) ;
#10134=ORIENTED_EDGE('',*,*,#7625,.T.) ;
#10135=ORIENTED_EDGE('',*,*,#7622,.T.) ;
#10136=ORIENTED_EDGE('',*,*,#7620,.F.) ;
#10137=ORIENTED_EDGE('',*,*,#7623,.F.) ;
#10138=ORIENTED_EDGE('',*,*,#7625,.F.) ;
#10139=ORIENTED_EDGE('',*,*,#7616,.F.) ;
#10140=ORIENTED_EDGE('',*,*,#7621,.F.) ;
#10141=ORIENTED_EDGE('',*,*,#7618,.F.) ;
#10142=ORIENTED_EDGE('',*,*,#7614,.F.) ;
#10143=ORIENTED_EDGE('',*,*,#7624,.F.) ;
#14676=ADVANCED_FACE('',(#1588,#651),#842,.F.) ;
#14677=ADVANCED_FACE('',(#1589),#1137,.F.) ;
#14678=ADVANCED_FACE('',(#1590),#1138,.F.) ;
#14679=ADVANCED_FACE('',(#1591,#652),#843,.F.) ;
#14680=ADVANCED_FACE('',(#1592),#1139,.F.) ;
#14681=ADVANCED_FACE('',(#1593),#1140,.F.) ;
#14682=ADVANCED_FACE('',(#1594,#653),#844,.F.) ;
#14683=ADVANCED_FACE('',(#1595),#1141,.F.) ;
#14684=ADVANCED_FACE('',(#1596),#1142,.F.) ;
#14685=ADVANCED_FACE('',(#1597,#654),#845,.F.) ;
#14686=ADVANCED_FACE('',(#1598),#1143,.F.) ;
#14687=ADVANCED_FACE('',(#1599),#1144,.F.) ;
#14688=ADVANCED_FACE('',(#1600,#655),#846,.F.) ;
#14689=ADVANCED_FACE('',(#1601),#1145,.F.) ;
#14690=ADVANCED_FACE('',(#1602),#1146,.F.) ;
#14691=ADVANCED_FACE('',(#1603,#656),#847,.F.) ;
#14692=ADVANCED_FACE('',(#1604),#1147,.F.) ;
#14693=ADVANCED_FACE('',(#1605),#1148,.F.) ;
#14694=ADVANCED_FACE('',(#1606,#657),#848,.F.) ;
#14695=ADVANCED_FACE('',(#1607),#1149,.F.) ;
#14696=ADVANCED_FACE('',(#1608),#1150,.F.) ;
#14697=ADVANCED_FACE('',(#1609,#658),#849,.F.) ;
#14698=ADVANCED_FACE('',(#1610),#1151,.F.) ;
#14699=ADVANCED_FACE('',(#1611),#1152,.F.) ;
#14700=ADVANCED_FACE('',(#1612,#659),#850,.F.) ;
#14701=ADVANCED_FACE('',(#1613),#1153,.F.) ;
#14702=ADVANCED_FACE('',(#1614),#1154,.F.) ;
#14703=ADVANCED_FACE('',(#1615,#660),#851,.F.) ;
#14704=ADVANCED_FACE('',(#1616),#1155,.F.) ;
#14705=ADVANCED_FACE('',(#1617),#1156,.F.) ;
#14706=ADVANCED_FACE('',(#1618,#661),#852,.F.) ;
#14707=ADVANCED_FACE('',(#1619),#1157,.F.) ;
#14708=ADVANCED_FACE('',(#1620),#1158,.F.) ;
#14709=ADVANCED_FACE('',(#1621,#662),#853,.F.) ;
#14710=ADVANCED_FACE('',(#1622),#1159,.F.) ;
#14711=ADVANCED_FACE('',(#1623),#1160,.F.) ;
#14712=ADVANCED_FACE('',(#1624,#663,#664,#665,#666,#667,#668,#669,#670,
#671,#672,#673,#674),#854,.T.) ;
#14713=ADVANCED_FACE('',(#1625),#855,.T.) ;
#14714=ADVANCED_FACE('',(#1626,#675,#676,#677,#678,#679,#680,#681,#682,
#683,#684,#685,#686),#856,.T.) ;
#14715=ADVANCED_FACE('',(#1627),#857,.T.) ;
#14716=ADVANCED_FACE('',(#1628),#858,.T.) ;
#14717=ADVANCED_FACE('',(#1629),#859,.T.) ;
#15495=CLOSED_SHELL('',(#14676,#14677,#14678,#14679,#14680,#14681,#14682,
#14683,#14684,#14685,#14686,#14687,#14688,#14689,#14690,#14691,#14692,#14693,
#14694,#14695,#14696,#14697,#14698,#14699,#14700,#14701,#14702,#14703,#14704,
#14705,#14706,#14707,#14708,#14709,#14710,#14711,#14712,#14713,#14714,#14715,
#14716,#14717)) ;
#15762=AXIS2_PLACEMENT_3D('',#23206,#18121,#18122) ;
#15763=AXIS2_PLACEMENT_3D('',#23207,#18123,#18124) ;
#15764=AXIS2_PLACEMENT_3D('',#23209,#18125,#18126) ;
#15765=AXIS2_PLACEMENT_3D('',#23211,#18127,#18128) ;
#15766=AXIS2_PLACEMENT_3D('',#23212,#18129,#18130) ;
#15767=AXIS2_PLACEMENT_3D('',#23214,#18131,#18132) ;
#15768=AXIS2_PLACEMENT_3D('',#23216,#18134,#18135) ;
#15769=AXIS2_PLACEMENT_3D('',#23219,#18137,#18138) ;
#15770=AXIS2_PLACEMENT_3D('',#23220,#18139,#18140) ;
#15771=AXIS2_PLACEMENT_3D('',#23222,#18141,#18142) ;
#15772=AXIS2_PLACEMENT_3D('',#23224,#18143,#18144) ;
#15773=AXIS2_PLACEMENT_3D('',#23225,#18145,#18146) ;
#15774=AXIS2_PLACEMENT_3D('',#23227,#18147,#18148) ;
#15775=AXIS2_PLACEMENT_3D('',#23229,#18150,#18151) ;
#15776=AXIS2_PLACEMENT_3D('',#23232,#18153,#18154) ;
#15777=AXIS2_PLACEMENT_3D('',#23233,#18155,#18156) ;
#15778=AXIS2_PLACEMENT_3D('',#23235,#18157,#18158) ;
#15779=AXIS2_PLACEMENT_3D('',#23237,#18159,#18160) ;
#15780=AXIS2_PLACEMENT_3D('',#23238,#18161,#18162) ;
#15781=AXIS2_PLACEMENT_3D('',#23240,#18163,#18164) ;
#15782=AXIS2_PLACEMENT_3D('',#23242,#18166,#18167) ;
#15783=AXIS2_PLACEMENT_3D('',#23245,#18169,#18170) ;
#15784=AXIS2_PLACEMENT_3D('',#23246,#18171,#18172) ;
#15785=AXIS2_PLACEMENT_3D('',#23248,#18173,#18174) ;
#15786=AXIS2_PLACEMENT_3D('',#23250,#18175,#18176) ;
#15787=AXIS2_PLACEMENT_3D('',#23251,#18177,#18178) ;
#15788=AXIS2_PLACEMENT_3D('',#23253,#18179,#18180) ;
#15789=AXIS2_PLACEMENT_3D('',#23255,#18182,#18183) ;
#15790=AXIS2_PLACEMENT_3D('',#23258,#18185,#18186) ;
#15791=AXIS2_PLACEMENT_3D('',#23259,#18187,#18188) ;
#15792=AXIS2_PLACEMENT_3D('',#23261,#18189,#18190) ;
#15793=AXIS2_PLACEMENT_3D('',#23263,#18191,#18192) ;
#15794=AXIS2_PLACEMENT_3D('',#23264,#18193,#18194) ;
#15795=AXIS2_PLACEMENT_3D('',#23266,#18195,#18196) ;
#15796=AXIS2_PLACEMENT_3D('',#23268,#18198,#18199) ;
#15797=AXIS2_PLACEMENT_3D('',#23271,#18201,#18202) ;
#15798=AXIS2_PLACEMENT_3D('',#23272,#18203,#18204) ;
#15799=AXIS2_PLACEMENT_3D('',#23274,#18205,#18206) ;
#15800=AXIS2_PLACEMENT_3D('',#23276,#18207,#18208) ;
#15801=AXIS2_PLACEMENT_3D('',#23277,#18209,#18210) ;
#15802=AXIS2_PLACEMENT_3D('',#23279,#18211,#18212) ;
#15803=AXIS2_PLACEMENT_3D('',#23281,#18214,#18215) ;
#15804=AXIS2_PLACEMENT_3D('',#23284,#18217,#18218) ;
#15805=AXIS2_PLACEMENT_3D('',#23285,#18219,#18220) ;
#15806=AXIS2_PLACEMENT_3D('',#23287,#18221,#18222) ;
#15807=AXIS2_PLACEMENT_3D('',#23289,#18223,#18224) ;
#15808=AXIS2_PLACEMENT_3D('',#23290,#18225,#18226) ;
#15809=AXIS2_PLACEMENT_3D('',#23292,#18227,#18228) ;
#15810=AXIS2_PLACEMENT_3D('',#23294,#18230,#18231) ;
#15811=AXIS2_PLACEMENT_3D('',#23297,#18233,#18234) ;
#15812=AXIS2_PLACEMENT_3D('',#23298,#18235,#18236) ;
#15813=AXIS2_PLACEMENT_3D('',#23300,#18237,#18238) ;
#15814=AXIS2_PLACEMENT_3D('',#23302,#18239,#18240) ;
#15815=AXIS2_PLACEMENT_3D('',#23303,#18241,#18242) ;
#15816=AXIS2_PLACEMENT_3D('',#23305,#18243,#18244) ;
#15817=AXIS2_PLACEMENT_3D('',#23307,#18246,#18247) ;
#15818=AXIS2_PLACEMENT_3D('',#23310,#18249,#18250) ;
#15819=AXIS2_PLACEMENT_3D('',#23311,#18251,#18252) ;
#15820=AXIS2_PLACEMENT_3D('',#23313,#18253,#18254) ;
#15821=AXIS2_PLACEMENT_3D('',#23315,#18255,#18256) ;
#15822=AXIS2_PLACEMENT_3D('',#23316,#18257,#18258) ;
#15823=AXIS2_PLACEMENT_3D('',#23318,#18259,#18260) ;
#15824=AXIS2_PLACEMENT_3D('',#23320,#18262,#18263) ;
#15825=AXIS2_PLACEMENT_3D('',#23323,#18265,#18266) ;
#15826=AXIS2_PLACEMENT_3D('',#23324,#18267,#18268) ;
#15827=AXIS2_PLACEMENT_3D('',#23326,#18269,#18270) ;
#15828=AXIS2_PLACEMENT_3D('',#23328,#18271,#18272) ;
#15829=AXIS2_PLACEMENT_3D('',#23329,#18273,#18274) ;
#15830=AXIS2_PLACEMENT_3D('',#23331,#18275,#18276) ;
#15831=AXIS2_PLACEMENT_3D('',#23333,#18278,#18279) ;
#15832=AXIS2_PLACEMENT_3D('',#23336,#18281,#18282) ;
#15833=AXIS2_PLACEMENT_3D('',#23337,#18283,#18284) ;
#15834=AXIS2_PLACEMENT_3D('',#23339,#18285,#18286) ;
#15835=AXIS2_PLACEMENT_3D('',#23341,#18287,#18288) ;
#15836=AXIS2_PLACEMENT_3D('',#23342,#18289,#18290) ;
#15837=AXIS2_PLACEMENT_3D('',#23344,#18291,#18292) ;
#15838=AXIS2_PLACEMENT_3D('',#23346,#18294,#18295) ;
#15839=AXIS2_PLACEMENT_3D('',#23349,#18297,#18298) ;
#15840=AXIS2_PLACEMENT_3D('',#23350,#18299,#18300) ;
#15841=AXIS2_PLACEMENT_3D('',#23352,#18301,#18302) ;
#15842=AXIS2_PLACEMENT_3D('',#23354,#18303,#18304) ;
#15843=AXIS2_PLACEMENT_3D('',#23355,#18305,#18306) ;
#15844=AXIS2_PLACEMENT_3D('',#23357,#18307,#18308) ;
#15845=AXIS2_PLACEMENT_3D('',#23359,#18310,#18311) ;
#15846=AXIS2_PLACEMENT_3D('',#23362,#18313,#18314) ;
#15847=AXIS2_PLACEMENT_3D('',#23363,#18315,#18316) ;
#15848=AXIS2_PLACEMENT_3D('',#23372,#18321,#18322) ;
#15849=AXIS2_PLACEMENT_3D('',#23378,#18326,#18327) ;
#15850=AXIS2_PLACEMENT_3D('',#23384,#18331,#18332) ;
#15851=AXIS2_PLACEMENT_3D('',#23387,#18335,#18336) ;
#15852=AXIS2_PLACEMENT_3D('',#23388,#18337,#18338) ;
#18121=DIRECTION('axis',(0.,0.,1.)) ;
#18122=DIRECTION('refdir',(1.,0.,0.)) ;
#18123=DIRECTION('center_axis',(3.5527136788005E-16,1.,0.)) ;
#18124=DIRECTION('ref_axis',(0.,0.,-1.)) ;
#18125=DIRECTION('center_axis',(3.5527136788005E-16,1.,0.)) ;
#18126=DIRECTION('ref_axis',(0.,0.,-1.)) ;
#18127=DIRECTION('center_axis',(3.5527136788005E-16,1.,0.)) ;
#18128=DIRECTION('ref_axis',(0.,0.,-1.)) ;
#18129=DIRECTION('center_axis',(3.5527136788005E-16,1.,0.)) ;
#18130=DIRECTION('ref_axis',(0.,0.,-1.)) ;
#18131=DIRECTION('center_axis',(3.5527136788005E-16,1.,0.)) ;
#18132=DIRECTION('ref_axis',(0.,0.,-1.)) ;
#18133=DIRECTION('',(3.5527136788005E-16,1.,0.)) ;
#18134=DIRECTION('center_axis',(3.5527136788005E-16,1.,0.)) ;
#18135=DIRECTION('ref_axis',(0.,0.,-1.)) ;
#18136=DIRECTION('',(3.5527136788005E-16,1.,0.)) ;
#18137=DIRECTION('center_axis',(-4.2632564145606E-15,-1.,0.)) ;
#18138=DIRECTION('ref_axis',(0.,0.,-1.)) ;
#18139=DIRECTION('center_axis',(3.5527136788005E-16,1.,0.)) ;
#18140=DIRECTION('ref_axis',(0.,0.,-1.)) ;
#18141=DIRECTION('center_axis',(3.5527136788005E-16,1.,0.)) ;
#18142=DIRECTION('ref_axis',(0.,0.,-1.)) ;
#18143=DIRECTION('center_axis',(3.5527136788005E-16,1.,0.)) ;
#18144=DIRECTION('ref_axis',(0.,0.,-1.)) ;
#18145=DIRECTION('center_axis',(3.5527136788005E-16,1.,0.)) ;
#18146=DIRECTION('ref_axis',(0.,0.,-1.)) ;
#18147=DIRECTION('center_axis',(3.5527136788005E-16,1.,0.)) ;
#18148=DIRECTION('ref_axis',(0.,0.,-1.)) ;
#18149=DIRECTION('',(3.5527136788005E-16,1.,0.)) ;
#18150=DIRECTION('center_axis',(3.5527136788005E-16,1.,0.)) ;
#18151=DIRECTION('ref_axis',(0.,0.,-1.)) ;
#18152=DIRECTION('',(3.5527136788005E-16,1.,0.)) ;
#18153=DIRECTION('center_axis',(-4.2632564145606E-15,-1.,0.)) ;
#18154=DIRECTION('ref_axis',(0.,0.,-1.)) ;
#18155=DIRECTION('center_axis',(3.5527136788005E-16,1.,0.)) ;
#18156=DIRECTION('ref_axis',(0.,0.,-1.)) ;
#18157=DIRECTION('center_axis',(3.5527136788005E-16,1.,0.)) ;
#18158=DIRECTION('ref_axis',(0.,0.,-1.)) ;
#18159=DIRECTION('center_axis',(3.5527136788005E-16,1.,0.)) ;
#18160=DIRECTION('ref_axis',(0.,0.,-1.)) ;
#18161=DIRECTION('center_axis',(3.5527136788005E-16,1.,0.)) ;
#18162=DIRECTION('ref_axis',(0.,0.,-1.)) ;
#18163=DIRECTION('center_axis',(3.5527136788005E-16,1.,0.)) ;
#18164=DIRECTION('ref_axis',(0.,0.,-1.)) ;
#18165=DIRECTION('',(3.5527136788005E-16,1.,0.)) ;
#18166=DIRECTION('center_axis',(3.5527136788005E-16,1.,0.)) ;
#18167=DIRECTION('ref_axis',(0.,0.,-1.)) ;
#18168=DIRECTION('',(3.5527136788005E-16,1.,0.)) ;
#18169=DIRECTION('center_axis',(-4.2632564145606E-15,-1.,0.)) ;
#18170=DIRECTION('ref_axis',(0.,0.,-1.)) ;
#18171=DIRECTION('center_axis',(3.5527136788005E-16,1.,0.)) ;
#18172=DIRECTION('ref_axis',(0.,0.,-1.)) ;
#18173=DIRECTION('center_axis',(3.5527136788005E-16,1.,0.)) ;
#18174=DIRECTION('ref_axis',(0.,0.,-1.)) ;
#18175=DIRECTION('center_axis',(3.5527136788005E-16,1.,0.)) ;
#18176=DIRECTION('ref_axis',(0.,0.,-1.)) ;
#18177=DIRECTION('center_axis',(3.5527136788005E-16,1.,0.)) ;
#18178=DIRECTION('ref_axis',(0.,0.,-1.)) ;
#18179=DIRECTION('center_axis',(3.5527136788005E-16,1.,0.)) ;
#18180=DIRECTION('ref_axis',(0.,0.,-1.)) ;
#18181=DIRECTION('',(3.5527136788005E-16,1.,0.)) ;
#18182=DIRECTION('center_axis',(3.5527136788005E-16,1.,0.)) ;
#18183=DIRECTION('ref_axis',(0.,0.,-1.)) ;
#18184=DIRECTION('',(3.5527136788005E-16,1.,0.)) ;
#18185=DIRECTION('center_axis',(-4.2632564145606E-15,-1.,0.)) ;
#18186=DIRECTION('ref_axis',(0.,0.,-1.)) ;
#18187=DIRECTION('center_axis',(3.5527136788005E-16,1.,0.)) ;
#18188=DIRECTION('ref_axis',(0.,0.,-1.)) ;
#18189=DIRECTION('center_axis',(3.5527136788005E-16,1.,0.)) ;
#18190=DIRECTION('ref_axis',(0.,0.,-1.)) ;
#18191=DIRECTION('center_axis',(3.5527136788005E-16,1.,0.)) ;
#18192=DIRECTION('ref_axis',(0.,0.,-1.)) ;
#18193=DIRECTION('center_axis',(3.5527136788005E-16,1.,0.)) ;
#18194=DIRECTION('ref_axis',(0.,0.,-1.)) ;
#18195=DIRECTION('center_axis',(3.5527136788005E-16,1.,0.)) ;
#18196=DIRECTION('ref_axis',(0.,0.,-1.)) ;
#18197=DIRECTION('',(3.5527136788005E-16,1.,0.)) ;
#18198=DIRECTION('center_axis',(3.5527136788005E-16,1.,0.)) ;
#18199=DIRECTION('ref_axis',(0.,0.,-1.)) ;
#18200=DIRECTION('',(3.5527136788005E-16,1.,0.)) ;
#18201=DIRECTION('center_axis',(-4.2632564145606E-15,-1.,0.)) ;
#18202=DIRECTION('ref_axis',(0.,0.,-1.)) ;
#18203=DIRECTION('center_axis',(3.5527136788005E-16,1.,0.)) ;
#18204=DIRECTION('ref_axis',(0.,0.,-1.)) ;
#18205=DIRECTION('center_axis',(3.5527136788005E-16,1.,0.)) ;
#18206=DIRECTION('ref_axis',(0.,0.,-1.)) ;
#18207=DIRECTION('center_axis',(3.5527136788005E-16,1.,0.)) ;
#18208=DIRECTION('ref_axis',(0.,0.,-1.)) ;
#18209=DIRECTION('center_axis',(3.5527136788005E-16,1.,0.)) ;
#18210=DIRECTION('ref_axis',(0.,0.,-1.)) ;
#18211=DIRECTION('center_axis',(3.5527136788005E-16,1.,0.)) ;
#18212=DIRECTION('ref_axis',(0.,0.,-1.)) ;
#18213=DIRECTION('',(3.5527136788005E-16,1.,0.)) ;
#18214=DIRECTION('center_axis',(3.5527136788005E-16,1.,0.)) ;
#18215=DIRECTION('ref_axis',(0.,0.,-1.)) ;
#18216=DIRECTION('',(3.5527136788005E-16,1.,0.)) ;
#18217=DIRECTION('center_axis',(-4.2632564145606E-15,-1.,0.)) ;
#18218=DIRECTION('ref_axis',(0.,0.,-1.)) ;
#18219=DIRECTION('center_axis',(3.5527136788005E-16,1.,0.)) ;
#18220=DIRECTION('ref_axis',(0.,0.,-1.)) ;
#18221=DIRECTION('center_axis',(3.5527136788005E-16,1.,0.)) ;
#18222=DIRECTION('ref_axis',(0.,0.,-1.)) ;
#18223=DIRECTION('center_axis',(3.5527136788005E-16,1.,0.)) ;
#18224=DIRECTION('ref_axis',(0.,0.,-1.)) ;
#18225=DIRECTION('center_axis',(3.5527136788005E-16,1.,0.)) ;
#18226=DIRECTION('ref_axis',(0.,0.,-1.)) ;
#18227=DIRECTION('center_axis',(3.5527136788005E-16,1.,0.)) ;
#18228=DIRECTION('ref_axis',(0.,0.,-1.)) ;
#18229=DIRECTION('',(3.5527136788005E-16,1.,0.)) ;
#18230=DIRECTION('center_axis',(3.5527136788005E-16,1.,0.)) ;
#18231=DIRECTION('ref_axis',(0.,0.,-1.)) ;
#18232=DIRECTION('',(3.5527136788005E-16,1.,0.)) ;
#18233=DIRECTION('center_axis',(-4.2632564145606E-15,-1.,0.)) ;
#18234=DIRECTION('ref_axis',(0.,0.,-1.)) ;
#18235=DIRECTION('center_axis',(3.5527136788005E-16,1.,0.)) ;
#18236=DIRECTION('ref_axis',(0.,0.,-1.)) ;
#18237=DIRECTION('center_axis',(3.5527136788005E-16,1.,0.)) ;
#18238=DIRECTION('ref_axis',(0.,0.,-1.)) ;
#18239=DIRECTION('center_axis',(3.5527136788005E-16,1.,0.)) ;
#18240=DIRECTION('ref_axis',(0.,0.,-1.)) ;
#18241=DIRECTION('center_axis',(3.5527136788005E-16,1.,0.)) ;
#18242=DIRECTION('ref_axis',(0.,0.,-1.)) ;
#18243=DIRECTION('center_axis',(3.5527136788005E-16,1.,0.)) ;
#18244=DIRECTION('ref_axis',(0.,0.,-1.)) ;
#18245=DIRECTION('',(3.5527136788005E-16,1.,0.)) ;
#18246=DIRECTION('center_axis',(3.5527136788005E-16,1.,0.)) ;
#18247=DIRECTION('ref_axis',(0.,0.,-1.)) ;
#18248=DIRECTION('',(3.5527136788005E-16,1.,0.)) ;
#18249=DIRECTION('center_axis',(-4.2632564145606E-15,-1.,0.)) ;
#18250=DIRECTION('ref_axis',(0.,0.,-1.)) ;
#18251=DIRECTION('center_axis',(1.77635683940025E-15,-1.,0.)) ;
#18252=DIRECTION('ref_axis',(0.,0.,1.)) ;
#18253=DIRECTION('center_axis',(1.77635683940025E-15,-1.,0.)) ;
#18254=DIRECTION('ref_axis',(0.,0.,1.)) ;
#18255=DIRECTION('center_axis',(1.77635683940025E-15,-1.,0.)) ;
#18256=DIRECTION('ref_axis',(0.,0.,1.)) ;
#18257=DIRECTION('center_axis',(1.77635683940025E-15,-1.,0.)) ;
#18258=DIRECTION('ref_axis',(0.,0.,1.)) ;
#18259=DIRECTION('center_axis',(-4.2632564145606E-15,-1.,0.)) ;
#18260=DIRECTION('ref_axis',(0.,0.,1.)) ;
#18261=DIRECTION('',(1.77635683940025E-15,-1.,0.)) ;
#18262=DIRECTION('center_axis',(1.77635683940025E-15,-1.,0.)) ;
#18263=DIRECTION('ref_axis',(0.,0.,1.)) ;
#18264=DIRECTION('',(1.77635683940025E-15,-1.,0.)) ;
#18265=DIRECTION('center_axis',(3.5527136788005E-16,1.,0.)) ;
#18266=DIRECTION('ref_axis',(0.,0.,1.)) ;
#18267=DIRECTION('center_axis',(1.77635683940025E-15,-1.,0.)) ;
#18268=DIRECTION('ref_axis',(0.,0.,1.)) ;
#18269=DIRECTION('center_axis',(1.77635683940025E-15,-1.,0.)) ;
#18270=DIRECTION('ref_axis',(0.,0.,1.)) ;
#18271=DIRECTION('center_axis',(1.77635683940025E-15,-1.,0.)) ;
#18272=DIRECTION('ref_axis',(0.,0.,1.)) ;
#18273=DIRECTION('center_axis',(1.77635683940025E-15,-1.,0.)) ;
#18274=DIRECTION('ref_axis',(0.,0.,1.)) ;
#18275=DIRECTION('center_axis',(-4.2632564145606E-15,-1.,0.)) ;
#18276=DIRECTION('ref_axis',(0.,0.,1.)) ;
#18277=DIRECTION('',(1.77635683940025E-15,-1.,0.)) ;
#18278=DIRECTION('center_axis',(1.77635683940025E-15,-1.,0.)) ;
#18279=DIRECTION('ref_axis',(0.,0.,1.)) ;
#18280=DIRECTION('',(1.77635683940025E-15,-1.,0.)) ;
#18281=DIRECTION('center_axis',(3.5527136788005E-16,1.,0.)) ;
#18282=DIRECTION('ref_axis',(0.,0.,1.)) ;
#18283=DIRECTION('center_axis',(1.77635683940025E-15,-1.,0.)) ;
#18284=DIRECTION('ref_axis',(0.,0.,1.)) ;
#18285=DIRECTION('center_axis',(1.77635683940025E-15,-1.,0.)) ;
#18286=DIRECTION('ref_axis',(0.,0.,1.)) ;
#18287=DIRECTION('center_axis',(1.77635683940025E-15,-1.,0.)) ;
#18288=DIRECTION('ref_axis',(0.,0.,1.)) ;
#18289=DIRECTION('center_axis',(1.77635683940025E-15,-1.,0.)) ;
#18290=DIRECTION('ref_axis',(0.,0.,1.)) ;
#18291=DIRECTION('center_axis',(-4.2632564145606E-15,-1.,0.)) ;
#18292=DIRECTION('ref_axis',(0.,0.,1.)) ;
#18293=DIRECTION('',(1.77635683940025E-15,-1.,0.)) ;
#18294=DIRECTION('center_axis',(1.77635683940025E-15,-1.,0.)) ;
#18295=DIRECTION('ref_axis',(0.,0.,1.)) ;
#18296=DIRECTION('',(1.77635683940025E-15,-1.,0.)) ;
#18297=DIRECTION('center_axis',(3.5527136788005E-16,1.,0.)) ;
#18298=DIRECTION('ref_axis',(0.,0.,1.)) ;
#18299=DIRECTION('center_axis',(1.77635683940025E-15,-1.,0.)) ;
#18300=DIRECTION('ref_axis',(0.,0.,1.)) ;
#18301=DIRECTION('center_axis',(1.77635683940025E-15,-1.,0.)) ;
#18302=DIRECTION('ref_axis',(0.,0.,1.)) ;
#18303=DIRECTION('center_axis',(1.77635683940025E-15,-1.,0.)) ;
#18304=DIRECTION('ref_axis',(0.,0.,1.)) ;
#18305=DIRECTION('center_axis',(1.77635683940025E-15,-1.,0.)) ;
#18306=DIRECTION('ref_axis',(0.,0.,1.)) ;
#18307=DIRECTION('center_axis',(-4.2632564145606E-15,-1.,0.)) ;
#18308=DIRECTION('ref_axis',(0.,0.,1.)) ;
#18309=DIRECTION('',(1.77635683940025E-15,-1.,0.)) ;
#18310=DIRECTION('center_axis',(1.77635683940025E-15,-1.,0.)) ;
#18311=DIRECTION('ref_axis',(0.,0.,1.)) ;
#18312=DIRECTION('',(1.77635683940025E-15,-1.,0.)) ;
#18313=DIRECTION('center_axis',(3.5527136788005E-16,1.,0.)) ;
#18314=DIRECTION('ref_axis',(0.,0.,1.)) ;
#18315=DIRECTION('center_axis',(4.2632564145606E-15,1.,0.)) ;
#18316=DIRECTION('ref_axis',(1.,-4.2632564145606E-15,0.)) ;
#18317=DIRECTION('',(-1.,4.2632564145606E-15,0.)) ;
#18318=DIRECTION('',(0.,0.,-1.)) ;
#18319=DIRECTION('',(1.,-4.2632564145606E-15,0.)) ;
#18320=DIRECTION('',(0.,0.,-1.)) ;
#18321=DIRECTION('center_axis',(-1.,-7.10542735760106E-15,0.)) ;
#18322=DIRECTION('ref_axis',(-7.10542735760106E-15,1.,0.)) ;
#18323=DIRECTION('',(7.10542735760106E-15,-1.,0.)) ;
#18324=DIRECTION('',(0.,0.,-1.)) ;
#18325=DIRECTION('',(-7.10542735760106E-15,1.,0.)) ;
#18326=DIRECTION('center_axis',(-3.5527136788005E-16,-1.,0.)) ;
#18327=DIRECTION('ref_axis',(-1.,3.5527136788005E-16,0.)) ;
#18328=DIRECTION('',(1.,-3.5527136788005E-16,0.)) ;
#18329=DIRECTION('',(0.,0.,-1.)) ;
#18330=DIRECTION('',(-1.,3.5527136788005E-16,0.)) ;
#18331=DIRECTION('center_axis',(1.,8.88178419700168E-16,0.)) ;
#18332=DIRECTION('ref_axis',(8.88178419700168E-16,-1.,0.)) ;
#18333=DIRECTION('',(-8.88178419700168E-16,1.,0.)) ;
#18334=DIRECTION('',(8.88178419700168E-16,-1.,0.)) ;
#18335=DIRECTION('center_axis',(0.,0.,1.)) ;
#18336=DIRECTION('ref_axis',(1.,0.,0.)) ;
#18337=DIRECTION('center_axis',(0.,0.,-1.)) ;
#18338=DIRECTION('ref_axis',(-1.,0.,0.)) ;
#23206=CARTESIAN_POINT('',(0.,0.,0.)) ;
#23207=CARTESIAN_POINT('Origin',(-63.0000000000005,199.45,-124.)) ;
#23208=CARTESIAN_POINT('',(-63.0000000000005,199.45,-115.)) ;
#23209=CARTESIAN_POINT('Origin',(-63.0000000000005,199.45,-124.)) ;
#23210=CARTESIAN_POINT('',(-63.0000000000005,199.45,-118.5)) ;
#23211=CARTESIAN_POINT('Origin',(-63.0000000000005,199.45,-124.)) ;
#23212=CARTESIAN_POINT('Origin',(-63.0000000000005,194.45,-124.)) ;
#23213=CARTESIAN_POINT('',(-63.0000000000005,189.45,-115.)) ;
#23214=CARTESIAN_POINT('Origin',(-63.0000000000005,189.45,-124.)) ;
#23215=CARTESIAN_POINT('',(-63.0000000000005,194.45,-115.)) ;
#23216=CARTESIAN_POINT('Origin',(-63.0000000000005,208.45,-124.)) ;
#23217=CARTESIAN_POINT('',(-63.0000000000005,209.45,-118.5)) ;
#23218=CARTESIAN_POINT('',(-63.0000000000005,208.45,-118.5)) ;
#23219=CARTESIAN_POINT('Origin',(-63.0000000000005,209.45,-124.)) ;
#23220=CARTESIAN_POINT('Origin',(-44.9999999999999,199.45,-12.)) ;
#23221=CARTESIAN_POINT('',(-44.9999999999999,199.45,-3.)) ;
#23222=CARTESIAN_POINT('Origin',(-44.9999999999999,199.45,-12.)) ;
#23223=CARTESIAN_POINT('',(-44.9999999999999,199.45,-6.5)) ;
#23224=CARTESIAN_POINT('Origin',(-44.9999999999999,199.45,-12.)) ;
#23225=CARTESIAN_POINT('Origin',(-44.9999999999999,194.45,-12.)) ;
#23226=CARTESIAN_POINT('',(-44.9999999999999,189.45,-3.)) ;
#23227=CARTESIAN_POINT('Origin',(-44.9999999999999,189.45,-12.)) ;
#23228=CARTESIAN_POINT('',(-44.9999999999999,194.45,-3.)) ;
#23229=CARTESIAN_POINT('Origin',(-44.9999999999999,208.45,-12.)) ;
#23230=CARTESIAN_POINT('',(-44.9999999999999,209.45,-6.5)) ;
#23231=CARTESIAN_POINT('',(-44.9999999999999,208.45,-6.5)) ;
#23232=CARTESIAN_POINT('Origin',(-44.9999999999999,209.45,-12.)) ;
#23233=CARTESIAN_POINT('Origin',(62.9999999999994,199.45,-124.)) ;
#23234=CARTESIAN_POINT('',(62.9999999999994,199.45,-115.)) ;
#23235=CARTESIAN_POINT('Origin',(62.9999999999994,199.45,-124.)) ;
#23236=CARTESIAN_POINT('',(62.9999999999994,199.45,-118.5)) ;
#23237=CARTESIAN_POINT('Origin',(62.9999999999994,199.45,-124.)) ;
#23238=CARTESIAN_POINT('Origin',(62.9999999999994,194.45,-124.)) ;
#23239=CARTESIAN_POINT('',(62.9999999999994,189.45,-115.)) ;
#23240=CARTESIAN_POINT('Origin',(62.9999999999994,189.45,-124.)) ;
#23241=CARTESIAN_POINT('',(62.9999999999994,194.45,-115.)) ;
#23242=CARTESIAN_POINT('Origin',(62.9999999999994,208.45,-124.)) ;
#23243=CARTESIAN_POINT('',(62.9999999999994,209.45,-118.5)) ;
#23244=CARTESIAN_POINT('',(62.9999999999994,208.45,-118.5)) ;
#23245=CARTESIAN_POINT('Origin',(62.9999999999994,209.45,-124.)) ;
#23246=CARTESIAN_POINT('Origin',(44.9999999999995,199.45,-12.)) ;
#23247=CARTESIAN_POINT('',(44.9999999999995,199.45,-3.)) ;
#23248=CARTESIAN_POINT('Origin',(44.9999999999995,199.45,-12.)) ;
#23249=CARTESIAN_POINT('',(44.9999999999995,199.45,-6.5)) ;
#23250=CARTESIAN_POINT('Origin',(44.9999999999995,199.45,-12.)) ;
#23251=CARTESIAN_POINT('Origin',(44.9999999999995,194.45,-12.)) ;
#23252=CARTESIAN_POINT('',(44.9999999999995,189.45,-3.)) ;
#23253=CARTESIAN_POINT('Origin',(44.9999999999995,189.45,-12.)) ;
#23254=CARTESIAN_POINT('',(44.9999999999995,194.45,-3.)) ;
#23255=CARTESIAN_POINT('Origin',(44.9999999999995,208.45,-12.)) ;
#23256=CARTESIAN_POINT('',(44.9999999999995,209.45,-6.5)) ;
#23257=CARTESIAN_POINT('',(44.9999999999995,208.45,-6.5)) ;
#23258=CARTESIAN_POINT('Origin',(44.9999999999995,209.45,-12.)) ;
#23259=CARTESIAN_POINT('Origin',(62.9999999999994,199.45,-54.)) ;
#23260=CARTESIAN_POINT('',(62.9999999999994,199.45,-45.)) ;
#23261=CARTESIAN_POINT('Origin',(62.9999999999994,199.45,-54.)) ;
#23262=CARTESIAN_POINT('',(62.9999999999994,199.45,-48.5)) ;
#23263=CARTESIAN_POINT('Origin',(62.9999999999994,199.45,-54.)) ;
#23264=CARTESIAN_POINT('Origin',(62.9999999999994,194.45,-54.)) ;
#23265=CARTESIAN_POINT('',(62.9999999999994,189.45,-45.)) ;
#23266=CARTESIAN_POINT('Origin',(62.9999999999994,189.45,-54.)) ;
#23267=CARTESIAN_POINT('',(62.9999999999994,194.45,-45.)) ;
#23268=CARTESIAN_POINT('Origin',(62.9999999999994,208.45,-54.)) ;
#23269=CARTESIAN_POINT('',(62.9999999999994,209.45,-48.5)) ;
#23270=CARTESIAN_POINT('',(62.9999999999994,208.45,-48.5)) ;
#23271=CARTESIAN_POINT('Origin',(62.9999999999994,209.45,-54.)) ;
#23272=CARTESIAN_POINT('Origin',(44.9999999999995,199.45,-166.)) ;
#23273=CARTESIAN_POINT('',(44.9999999999995,199.45,-157.)) ;
#23274=CARTESIAN_POINT('Origin',(44.9999999999995,199.45,-166.)) ;
#23275=CARTESIAN_POINT('',(44.9999999999995,199.45,-160.5)) ;
#23276=CARTESIAN_POINT('Origin',(44.9999999999995,199.45,-166.)) ;
#23277=CARTESIAN_POINT('Origin',(44.9999999999995,194.45,-166.)) ;
#23278=CARTESIAN_POINT('',(44.9999999999995,189.45,-157.)) ;
#23279=CARTESIAN_POINT('Origin',(44.9999999999995,189.45,-166.)) ;
#23280=CARTESIAN_POINT('',(44.9999999999995,194.45,-157.)) ;
#23281=CARTESIAN_POINT('Origin',(44.9999999999995,208.45,-166.)) ;
#23282=CARTESIAN_POINT('',(44.9999999999995,209.45,-160.5)) ;
#23283=CARTESIAN_POINT('',(44.9999999999995,208.45,-160.5)) ;
#23284=CARTESIAN_POINT('Origin',(44.9999999999995,209.45,-166.)) ;
#23285=CARTESIAN_POINT('Origin',(-63.0000000000005,199.45,-54.)) ;
#23286=CARTESIAN_POINT('',(-63.0000000000005,199.45,-45.)) ;
#23287=CARTESIAN_POINT('Origin',(-63.0000000000005,199.45,-54.)) ;
#23288=CARTESIAN_POINT('',(-63.0000000000005,199.45,-48.5)) ;
#23289=CARTESIAN_POINT('Origin',(-63.0000000000005,199.45,-54.)) ;
#23290=CARTESIAN_POINT('Origin',(-63.0000000000005,194.45,-54.)) ;
#23291=CARTESIAN_POINT('',(-63.0000000000005,189.45,-45.)) ;
#23292=CARTESIAN_POINT('Origin',(-63.0000000000005,189.45,-54.)) ;
#23293=CARTESIAN_POINT('',(-63.0000000000005,194.45,-45.)) ;
#23294=CARTESIAN_POINT('Origin',(-63.0000000000005,208.45,-54.)) ;
#23295=CARTESIAN_POINT('',(-63.0000000000005,209.45,-48.5)) ;
#23296=CARTESIAN_POINT('',(-63.0000000000005,208.45,-48.5)) ;
#23297=CARTESIAN_POINT('Origin',(-63.0000000000005,209.45,-54.)) ;
#23298=CARTESIAN_POINT('Origin',(-44.9999999999999,199.45,-166.)) ;
#23299=CARTESIAN_POINT('',(-44.9999999999999,199.45,-157.)) ;
#23300=CARTESIAN_POINT('Origin',(-44.9999999999999,199.45,-166.)) ;
#23301=CARTESIAN_POINT('',(-44.9999999999999,199.45,-160.5)) ;
#23302=CARTESIAN_POINT('Origin',(-44.9999999999999,199.45,-166.)) ;
#23303=CARTESIAN_POINT('Origin',(-44.9999999999999,194.45,-166.)) ;
#23304=CARTESIAN_POINT('',(-44.9999999999999,189.45,-157.)) ;
#23305=CARTESIAN_POINT('Origin',(-44.9999999999999,189.45,-166.)) ;
#23306=CARTESIAN_POINT('',(-44.9999999999999,194.45,-157.)) ;
#23307=CARTESIAN_POINT('Origin',(-44.9999999999999,208.45,-166.)) ;
#23308=CARTESIAN_POINT('',(-44.9999999999999,209.45,-160.5)) ;
#23309=CARTESIAN_POINT('',(-44.9999999999999,208.45,-160.5)) ;
#23310=CARTESIAN_POINT('Origin',(-44.9999999999999,209.45,-166.)) ;
#23311=CARTESIAN_POINT('Origin',(-87.4999999999996,199.449999999999,-158.)) ;
#23312=CARTESIAN_POINT('',(-87.4999999999996,199.449999999999,-167.)) ;
#23313=CARTESIAN_POINT('Origin',(-87.4999999999996,199.449999999999,-158.)) ;
#23314=CARTESIAN_POINT('',(-87.4999999999996,199.449999999999,-163.5)) ;
#23315=CARTESIAN_POINT('Origin',(-87.4999999999996,199.449999999999,-158.)) ;
#23316=CARTESIAN_POINT('Origin',(-87.4999999999996,204.449999999999,-158.)) ;
#23317=CARTESIAN_POINT('',(-87.4999999999996,209.45,-167.)) ;
#23318=CARTESIAN_POINT('Origin',(-87.4999999999996,209.45,-158.)) ;
#23319=CARTESIAN_POINT('',(-87.4999999999996,204.449999999999,-167.)) ;
#23320=CARTESIAN_POINT('Origin',(-87.4999999999996,189.449999999999,-158.)) ;
#23321=CARTESIAN_POINT('',(-87.4999999999996,189.45,-163.5)) ;
#23322=CARTESIAN_POINT('',(-87.4999999999996,189.449999999999,-163.5)) ;
#23323=CARTESIAN_POINT('Origin',(-87.4999999999996,189.45,-158.)) ;
#23324=CARTESIAN_POINT('Origin',(87.5000000000001,199.45,-20.)) ;
#23325=CARTESIAN_POINT('',(87.5000000000001,199.45,-29.)) ;
#23326=CARTESIAN_POINT('Origin',(87.5000000000001,199.45,-20.)) ;
#23327=CARTESIAN_POINT('',(87.5000000000001,199.45,-25.5)) ;
#23328=CARTESIAN_POINT('Origin',(87.5000000000001,199.45,-20.)) ;
#23329=CARTESIAN_POINT('Origin',(87.5000000000001,204.45,-20.)) ;
#23330=CARTESIAN_POINT('',(87.5000000000001,209.45,-29.)) ;
#23331=CARTESIAN_POINT('Origin',(87.5000000000001,209.45,-20.)) ;
#23332=CARTESIAN_POINT('',(87.5000000000001,204.45,-29.)) ;
#23333=CARTESIAN_POINT('Origin',(87.5000000000001,189.45,-20.)) ;
#23334=CARTESIAN_POINT('',(87.5000000000001,189.45,-25.5)) ;
#23335=CARTESIAN_POINT('',(87.5000000000001,189.45,-25.5)) ;
#23336=CARTESIAN_POINT('Origin',(87.5000000000001,189.45,-20.)) ;
#23337=CARTESIAN_POINT('Origin',(87.5000000000001,199.45,-158.)) ;
#23338=CARTESIAN_POINT('',(87.5000000000001,199.45,-167.)) ;
#23339=CARTESIAN_POINT('Origin',(87.5000000000001,199.45,-158.)) ;
#23340=CARTESIAN_POINT('',(87.5000000000001,199.45,-163.5)) ;
#23341=CARTESIAN_POINT('Origin',(87.5000000000001,199.45,-158.)) ;
#23342=CARTESIAN_POINT('Origin',(87.5000000000001,204.45,-158.)) ;
#23343=CARTESIAN_POINT('',(87.5,209.45,-167.)) ;
#23344=CARTESIAN_POINT('Origin',(87.5,209.45,-158.)) ;
#23345=CARTESIAN_POINT('',(87.5000000000001,204.45,-167.)) ;
#23346=CARTESIAN_POINT('Origin',(87.5000000000001,189.45,-158.)) ;
#23347=CARTESIAN_POINT('',(87.5000000000001,189.45,-163.5)) ;
#23348=CARTESIAN_POINT('',(87.5000000000001,189.45,-163.5)) ;
#23349=CARTESIAN_POINT('Origin',(87.5000000000001,189.45,-158.)) ;
#23350=CARTESIAN_POINT('Origin',(-87.4999999999996,199.449999999999,-20.)) ;
#23351=CARTESIAN_POINT('',(-87.4999999999996,199.449999999999,-29.)) ;
#23352=CARTESIAN_POINT('Origin',(-87.4999999999996,199.449999999999,-20.)) ;
#23353=CARTESIAN_POINT('',(-87.4999999999996,199.449999999999,-25.5)) ;
#23354=CARTESIAN_POINT('Origin',(-87.4999999999996,199.449999999999,-20.)) ;
#23355=CARTESIAN_POINT('Origin',(-87.4999999999996,204.449999999999,-20.)) ;
#23356=CARTESIAN_POINT('',(-87.4999999999996,209.45,-29.)) ;
#23357=CARTESIAN_POINT('Origin',(-87.4999999999996,209.45,-20.)) ;
#23358=CARTESIAN_POINT('',(-87.4999999999996,204.449999999999,-29.)) ;
#23359=CARTESIAN_POINT('Origin',(-87.4999999999995,189.449999999999,-20.)) ;
#23360=CARTESIAN_POINT('',(-87.4999999999995,189.45,-25.5)) ;
#23361=CARTESIAN_POINT('',(-87.4999999999995,189.449999999999,-25.5)) ;
#23362=CARTESIAN_POINT('Origin',(-87.4999999999995,189.45,-20.)) ;
#23363=CARTESIAN_POINT('Origin',(-100.,209.45,0.)) ;
#23364=CARTESIAN_POINT('',(100.,209.449999999999,-178.)) ;
#23365=CARTESIAN_POINT('',(-100.,209.45,-178.)) ;
#23366=CARTESIAN_POINT('',(-50.0000000000001,209.45,-178.)) ;
#23367=CARTESIAN_POINT('',(-100.,209.45,0.)) ;
#23368=CARTESIAN_POINT('',(-100.,209.45,0.)) ;
#23369=CARTESIAN_POINT('',(100.,209.449999999999,0.)) ;
#23370=CARTESIAN_POINT('',(-100.,209.45,0.)) ;
#23371=CARTESIAN_POINT('',(100.,209.449999999999,0.)) ;
#23372=CARTESIAN_POINT('Origin',(-100.,189.45,0.)) ;
#23373=CARTESIAN_POINT('',(-100.,189.45,-178.)) ;
#23374=CARTESIAN_POINT('',(-100.,194.45,-178.)) ;
#23375=CARTESIAN_POINT('',(-100.,189.45,0.)) ;
#23376=CARTESIAN_POINT('',(-100.,189.45,0.)) ;
#23377=CARTESIAN_POINT('',(-100.,189.45,0.)) ;
#23378=CARTESIAN_POINT('Origin',(100.,189.45,0.)) ;
#23379=CARTESIAN_POINT('',(100.,189.45,-178.)) ;
#23380=CARTESIAN_POINT('',(50.,189.45,-178.)) ;
#23381=CARTESIAN_POINT('',(100.,189.45,0.)) ;
#23382=CARTESIAN_POINT('',(100.,189.45,0.)) ;
#23383=CARTESIAN_POINT('',(100.,189.45,0.)) ;
#23384=CARTESIAN_POINT('Origin',(100.,209.449999999999,0.)) ;
#23385=CARTESIAN_POINT('',(100.,204.45,-178.)) ;
#23386=CARTESIAN_POINT('',(100.,209.449999999999,0.)) ;
#23387=CARTESIAN_POINT('Origin',(-3.5527136788005E-14,199.45,0.)) ;
#23388=CARTESIAN_POINT('Origin',(-4.44089209850063E-14,199.45,-178.)) ;
#63793=UNCERTAINTY_MEASURE_WITH_UNIT(LENGTH_MEASURE(0.01),#63825,
'DISTANCE_ACCURACY_VALUE',
'Maximum model space distance between geometric entities at asserted c
onnectivities') ;
#63807=UNCERTAINTY_MEASURE_WITH_UNIT(LENGTH_MEASURE(0.01),#63825,
'DISTANCE_ACCURACY_VALUE',
'Maximum model space distance between geometric entities at asserted c
onnectivities') ;
#63810=(
GEOMETRIC_REPRESENTATION_CONTEXT(3)
GLOBAL_UNCERTAINTY_ASSIGNED_CONTEXT((#63793))
GLOBAL_UNIT_ASSIGNED_CONTEXT((#63825,#63827,#63828))
REPRESENTATION_CONTEXT('','3D')
) ;
#63824=(
GEOMETRIC_REPRESENTATION_CONTEXT(3)
GLOBAL_UNCERTAINTY_ASSIGNED_CONTEXT((#63807))
GLOBAL_UNIT_ASSIGNED_CONTEXT((#63825,#63827,#63828))
REPRESENTATION_CONTEXT('','3D')
) ;
#63825=(
LENGTH_UNIT()
NAMED_UNIT(*)
SI_UNIT(.MILLI.,.METRE.)
) ;
#63827=(
NAMED_UNIT(*)
PLANE_ANGLE_UNIT()
SI_UNIT($,.RADIAN.)
) ;
#63828=(
NAMED_UNIT(*)
SI_UNIT($,.STERADIAN.)
SOLID_ANGLE_UNIT()
) ;
#63831=SHAPE_DEFINITION_REPRESENTATION(#63847,#63880) ;
#63847=PRODUCT_DEFINITION_SHAPE('',$,#63897) ;
#63880=SHAPE_REPRESENTATION('',(#15762),#63810) ;
#63894=PRODUCT_DEFINITION_CONTEXT('part definition',#63944,'design') ;
#63897=PRODUCT_DEFINITION('Bottom_Plate','Bottom_Plate',#63913,#63894) ;
#63913=PRODUCT_DEFINITION_FORMATION('',$,#63948) ;
#63944=APPLICATION_CONTEXT(
'Core Data for Automotive Mechanical Design Process') ;
#63945=PRODUCT_CONTEXT('part definition',#63944,'mechanical') ;
#63948=PRODUCT('Bottom_Plate','Bottom_Plate',$,(#63945)) ;
#63963=PRESENTATION_STYLE_ASSIGNMENT((#63968)) ;
#63968=SURFACE_STYLE_USAGE(.BOTH.,#63973) ;
#63973=SURFACE_SIDE_STYLE('',(#63978)) ;
#63978=SURFACE_STYLE_FILL_AREA(#63983) ;
#63983=FILL_AREA_STYLE('Opaque(160,160,160)',(#63988)) ;
#63988=FILL_AREA_STYLE_COLOUR('Opaque(160,160,160)',#63993) ;
#63993=COLOUR_RGB('Opaque(160,160,160)', 0.09019608, 0.27058824, 0.51372549) ;
ENDSEC;
END-ISO-10303-21;
